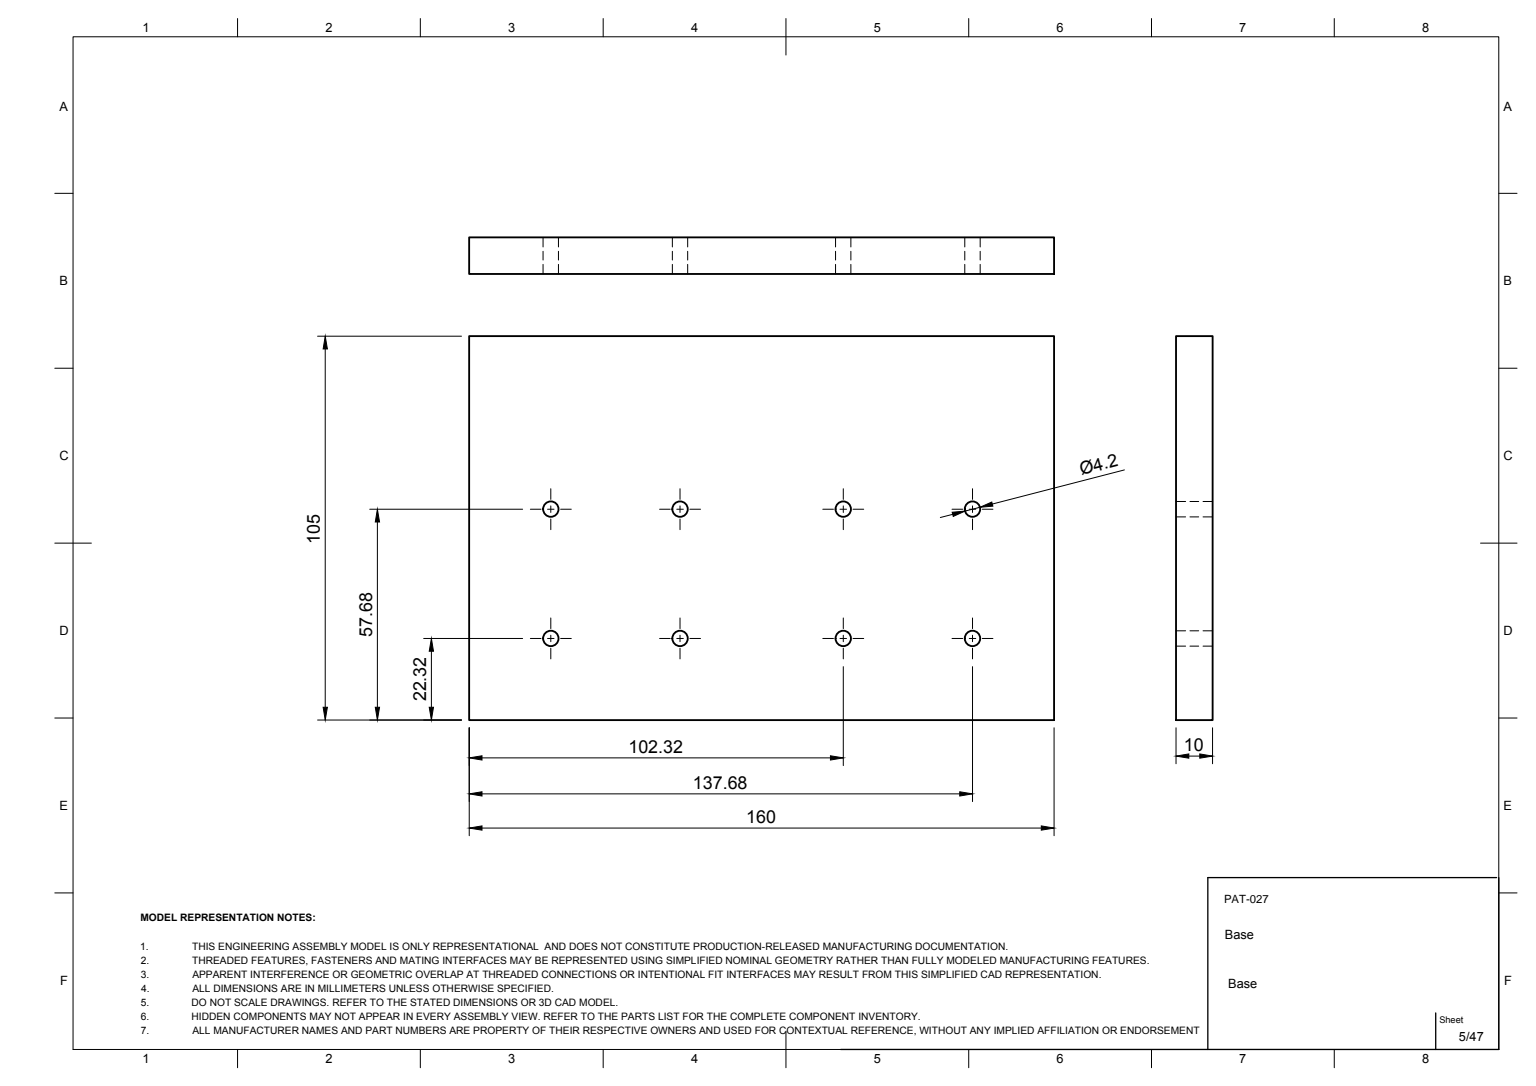
ISO-10303-21;
HEADER;
/* Generated by software containing ST-Developer
 * from STEP Tools, Inc. (www.steptools.com) 
 */

FILE_DESCRIPTION(
/* description */ ('Crank-driven oscillating fan base (mechanism only)'),

/* implementation_level */ '2;1');

FILE_NAME(
/* name */ 'Base.step',
/* time_stamp */ '2026-10-28T03:25:00-07:00',
/* author */ (''),
/* organization */ (''),
/* preprocessor_version */ 'ST-DEVELOPER v20.2',
/* originating_system */ 'Autodesk Translation Framework v15.17.0.0',
/* authorisation */ '');

FILE_SCHEMA (('AUTOMOTIVE_DESIGN { 1 0 10303 214 3 1 1 }'));
ENDSEC;

DATA;
#10=MECHANICAL_DESIGN_GEOMETRIC_PRESENTATION_REPRESENTATION('',(#437),#11916);
#357=SHAPE_REPRESENTATION_RELATIONSHIP('SRR','None',#12081,#397);
#397=ADVANCED_BREP_SHAPE_REPRESENTATION('',(#485),#11872);
#437=STYLED_ITEM('',(#12354),#485);
#485=MANIFOLD_SOLID_BREP('Body1',#6067);
#530=FACE_BOUND('',#1274,.T.);
#531=FACE_BOUND('',#1275,.T.);
#532=FACE_BOUND('',#1276,.T.);
#533=FACE_BOUND('',#1277,.T.);
#534=FACE_BOUND('',#1278,.T.);
#535=FACE_BOUND('',#1279,.T.);
#536=FACE_BOUND('',#1280,.T.);
#537=FACE_BOUND('',#1281,.T.);
#538=FACE_BOUND('',#1283,.T.);
#539=FACE_BOUND('',#1284,.T.);
#540=FACE_BOUND('',#1285,.T.);
#541=FACE_BOUND('',#1286,.T.);
#542=FACE_BOUND('',#1287,.T.);
#543=FACE_BOUND('',#1288,.T.);
#544=FACE_BOUND('',#1289,.T.);
#545=FACE_BOUND('',#1290,.T.);
#692=PLANE('',#6586);
#693=PLANE('',#6587);
#694=PLANE('',#6588);
#695=PLANE('',#6589);
#696=PLANE('',#6590);
#697=PLANE('',#6591);
#886=FACE_OUTER_BOUND('',#1261,.T.);
#887=FACE_OUTER_BOUND('',#1262,.T.);
#888=FACE_OUTER_BOUND('',#1263,.T.);
#889=FACE_OUTER_BOUND('',#1264,.T.);
#890=FACE_OUTER_BOUND('',#1265,.T.);
#891=FACE_OUTER_BOUND('',#1266,.T.);
#892=FACE_OUTER_BOUND('',#1267,.T.);
#893=FACE_OUTER_BOUND('',#1268,.T.);
#894=FACE_OUTER_BOUND('',#1269,.T.);
#895=FACE_OUTER_BOUND('',#1270,.T.);
#896=FACE_OUTER_BOUND('',#1271,.T.);
#897=FACE_OUTER_BOUND('',#1272,.T.);
#898=FACE_OUTER_BOUND('',#1273,.T.);
#899=FACE_OUTER_BOUND('',#1282,.T.);
#1261=EDGE_LOOP('',(#4068,#4069,#4070,#4071));
#1262=EDGE_LOOP('',(#4072,#4073,#4074,#4075));
#1263=EDGE_LOOP('',(#4076,#4077,#4078,#4079));
#1264=EDGE_LOOP('',(#4080,#4081,#4082,#4083));
#1265=EDGE_LOOP('',(#4084,#4085,#4086,#4087));
#1266=EDGE_LOOP('',(#4088,#4089,#4090,#4091));
#1267=EDGE_LOOP('',(#4092,#4093,#4094,#4095));
#1268=EDGE_LOOP('',(#4096,#4097,#4098,#4099));
#1269=EDGE_LOOP('',(#4100,#4101,#4102,#4103));
#1270=EDGE_LOOP('',(#4104,#4105,#4106,#4107));
#1271=EDGE_LOOP('',(#4108,#4109,#4110,#4111));
#1272=EDGE_LOOP('',(#4112,#4113,#4114,#4115));
#1273=EDGE_LOOP('',(#4116,#4117,#4118,#4119));
#1274=EDGE_LOOP('',(#4120));
#1275=EDGE_LOOP('',(#4121));
#1276=EDGE_LOOP('',(#4122));
#1277=EDGE_LOOP('',(#4123));
#1278=EDGE_LOOP('',(#4124));
#1279=EDGE_LOOP('',(#4125));
#1280=EDGE_LOOP('',(#4126));
#1281=EDGE_LOOP('',(#4127));
#1282=EDGE_LOOP('',(#4128,#4129,#4130,#4131));
#1283=EDGE_LOOP('',(#4132));
#1284=EDGE_LOOP('',(#4133));
#1285=EDGE_LOOP('',(#4134));
#1286=EDGE_LOOP('',(#4135));
#1287=EDGE_LOOP('',(#4136));
#1288=EDGE_LOOP('',(#4137));
#1289=EDGE_LOOP('',(#4138));
#1290=EDGE_LOOP('',(#4139));
#1798=LINE('',#9455,#2131);
#1799=LINE('',#9461,#2132);
#1800=LINE('',#9467,#2133);
#1801=LINE('',#9473,#2134);
#1802=LINE('',#9479,#2135);
#1803=LINE('',#9485,#2136);
#1804=LINE('',#9491,#2137);
#1805=LINE('',#9497,#2138);
#1806=LINE('',#9502,#2139);
#1807=LINE('',#9504,#2140);
#1808=LINE('',#9506,#2141);
#1809=LINE('',#9507,#2142);
#1810=LINE('',#9510,#2143);
#1811=LINE('',#9512,#2144);
#1812=LINE('',#9513,#2145);
#1813=LINE('',#9516,#2146);
#1814=LINE('',#9518,#2147);
#1815=LINE('',#9519,#2148);
#1816=LINE('',#9521,#2149);
#1817=LINE('',#9522,#2150);
#2131=VECTOR('',#7421,0.21);
#2132=VECTOR('',#7428,0.21);
#2133=VECTOR('',#7435,0.210000000000001);
#2134=VECTOR('',#7442,0.210000000000001);
#2135=VECTOR('',#7449,0.21);
#2136=VECTOR('',#7456,0.21);
#2137=VECTOR('',#7463,0.21);
#2138=VECTOR('',#7470,0.21);
#2139=VECTOR('',#7475,1.);
#2140=VECTOR('',#7476,1.);
#2141=VECTOR('',#7477,1.);
#2142=VECTOR('',#7478,1.);
#2143=VECTOR('',#7481,1.);
#2144=VECTOR('',#7482,1.);
#2145=VECTOR('',#7483,1.);
#2146=VECTOR('',#7486,1.);
#2147=VECTOR('',#7487,1.);
#2148=VECTOR('',#7488,1.);
#2149=VECTOR('',#7491,1.);
#2150=VECTOR('',#7492,1.);
#2464=CIRCLE('',#6563,0.21);
#2465=CIRCLE('',#6564,0.21);
#2466=CIRCLE('',#6566,0.21);
#2467=CIRCLE('',#6567,0.21);
#2468=CIRCLE('',#6569,0.210000000000001);
#2469=CIRCLE('',#6570,0.210000000000001);
#2470=CIRCLE('',#6572,0.210000000000001);
#2471=CIRCLE('',#6573,0.210000000000001);
#2472=CIRCLE('',#6575,0.21);
#2473=CIRCLE('',#6576,0.21);
#2474=CIRCLE('',#6578,0.21);
#2475=CIRCLE('',#6579,0.21);
#2476=CIRCLE('',#6581,0.21);
#2477=CIRCLE('',#6582,0.21);
#2478=CIRCLE('',#6584,0.21);
#2479=CIRCLE('',#6585,0.21);
#2829=VERTEX_POINT('',#9452);
#2830=VERTEX_POINT('',#9454);
#2831=VERTEX_POINT('',#9458);
#2832=VERTEX_POINT('',#9460);
#2833=VERTEX_POINT('',#9464);
#2834=VERTEX_POINT('',#9466);
#2835=VERTEX_POINT('',#9470);
#2836=VERTEX_POINT('',#9472);
#2837=VERTEX_POINT('',#9476);
#2838=VERTEX_POINT('',#9478);
#2839=VERTEX_POINT('',#9482);
#2840=VERTEX_POINT('',#9484);
#2841=VERTEX_POINT('',#9488);
#2842=VERTEX_POINT('',#9490);
#2843=VERTEX_POINT('',#9494);
#2844=VERTEX_POINT('',#9496);
#2845=VERTEX_POINT('',#9500);
#2846=VERTEX_POINT('',#9501);
#2847=VERTEX_POINT('',#9503);
#2848=VERTEX_POINT('',#9505);
#2849=VERTEX_POINT('',#9509);
#2850=VERTEX_POINT('',#9511);
#2851=VERTEX_POINT('',#9515);
#2852=VERTEX_POINT('',#9517);
#3329=EDGE_CURVE('',#2829,#2829,#2464,.T.);
#3330=EDGE_CURVE('',#2829,#2830,#1798,.T.);
#3331=EDGE_CURVE('',#2830,#2830,#2465,.T.);
#3332=EDGE_CURVE('',#2831,#2831,#2466,.T.);
#3333=EDGE_CURVE('',#2831,#2832,#1799,.T.);
#3334=EDGE_CURVE('',#2832,#2832,#2467,.T.);
#3335=EDGE_CURVE('',#2833,#2833,#2468,.T.);
#3336=EDGE_CURVE('',#2833,#2834,#1800,.T.);
#3337=EDGE_CURVE('',#2834,#2834,#2469,.T.);
#3338=EDGE_CURVE('',#2835,#2835,#2470,.T.);
#3339=EDGE_CURVE('',#2835,#2836,#1801,.T.);
#3340=EDGE_CURVE('',#2836,#2836,#2471,.T.);
#3341=EDGE_CURVE('',#2837,#2837,#2472,.T.);
#3342=EDGE_CURVE('',#2837,#2838,#1802,.T.);
#3343=EDGE_CURVE('',#2838,#2838,#2473,.T.);
#3344=EDGE_CURVE('',#2839,#2839,#2474,.T.);
#3345=EDGE_CURVE('',#2839,#2840,#1803,.T.);
#3346=EDGE_CURVE('',#2840,#2840,#2475,.T.);
#3347=EDGE_CURVE('',#2841,#2841,#2476,.T.);
#3348=EDGE_CURVE('',#2841,#2842,#1804,.T.);
#3349=EDGE_CURVE('',#2842,#2842,#2477,.T.);
#3350=EDGE_CURVE('',#2843,#2843,#2478,.T.);
#3351=EDGE_CURVE('',#2843,#2844,#1805,.T.);
#3352=EDGE_CURVE('',#2844,#2844,#2479,.T.);
#3353=EDGE_CURVE('',#2845,#2846,#1806,.T.);
#3354=EDGE_CURVE('',#2846,#2847,#1807,.T.);
#3355=EDGE_CURVE('',#2848,#2847,#1808,.T.);
#3356=EDGE_CURVE('',#2845,#2848,#1809,.T.);
#3357=EDGE_CURVE('',#2849,#2845,#1810,.T.);
#3358=EDGE_CURVE('',#2850,#2848,#1811,.T.);
#3359=EDGE_CURVE('',#2849,#2850,#1812,.T.);
#3360=EDGE_CURVE('',#2851,#2849,#1813,.T.);
#3361=EDGE_CURVE('',#2852,#2850,#1814,.T.);
#3362=EDGE_CURVE('',#2851,#2852,#1815,.T.);
#3363=EDGE_CURVE('',#2846,#2851,#1816,.T.);
#3364=EDGE_CURVE('',#2847,#2852,#1817,.T.);
#4068=ORIENTED_EDGE('',*,*,#3329,.F.);
#4069=ORIENTED_EDGE('',*,*,#3330,.T.);
#4070=ORIENTED_EDGE('',*,*,#3331,.F.);
#4071=ORIENTED_EDGE('',*,*,#3330,.F.);
#4072=ORIENTED_EDGE('',*,*,#3332,.F.);
#4073=ORIENTED_EDGE('',*,*,#3333,.T.);
#4074=ORIENTED_EDGE('',*,*,#3334,.F.);
#4075=ORIENTED_EDGE('',*,*,#3333,.F.);
#4076=ORIENTED_EDGE('',*,*,#3335,.F.);
#4077=ORIENTED_EDGE('',*,*,#3336,.T.);
#4078=ORIENTED_EDGE('',*,*,#3337,.F.);
#4079=ORIENTED_EDGE('',*,*,#3336,.F.);
#4080=ORIENTED_EDGE('',*,*,#3338,.F.);
#4081=ORIENTED_EDGE('',*,*,#3339,.T.);
#4082=ORIENTED_EDGE('',*,*,#3340,.F.);
#4083=ORIENTED_EDGE('',*,*,#3339,.F.);
#4084=ORIENTED_EDGE('',*,*,#3341,.F.);
#4085=ORIENTED_EDGE('',*,*,#3342,.T.);
#4086=ORIENTED_EDGE('',*,*,#3343,.F.);
#4087=ORIENTED_EDGE('',*,*,#3342,.F.);
#4088=ORIENTED_EDGE('',*,*,#3344,.F.);
#4089=ORIENTED_EDGE('',*,*,#3345,.T.);
#4090=ORIENTED_EDGE('',*,*,#3346,.F.);
#4091=ORIENTED_EDGE('',*,*,#3345,.F.);
#4092=ORIENTED_EDGE('',*,*,#3347,.F.);
#4093=ORIENTED_EDGE('',*,*,#3348,.T.);
#4094=ORIENTED_EDGE('',*,*,#3349,.F.);
#4095=ORIENTED_EDGE('',*,*,#3348,.F.);
#4096=ORIENTED_EDGE('',*,*,#3350,.F.);
#4097=ORIENTED_EDGE('',*,*,#3351,.T.);
#4098=ORIENTED_EDGE('',*,*,#3352,.F.);
#4099=ORIENTED_EDGE('',*,*,#3351,.F.);
#4100=ORIENTED_EDGE('',*,*,#3353,.T.);
#4101=ORIENTED_EDGE('',*,*,#3354,.T.);
#4102=ORIENTED_EDGE('',*,*,#3355,.F.);
#4103=ORIENTED_EDGE('',*,*,#3356,.F.);
#4104=ORIENTED_EDGE('',*,*,#3357,.T.);
#4105=ORIENTED_EDGE('',*,*,#3356,.T.);
#4106=ORIENTED_EDGE('',*,*,#3358,.F.);
#4107=ORIENTED_EDGE('',*,*,#3359,.F.);
#4108=ORIENTED_EDGE('',*,*,#3360,.T.);
#4109=ORIENTED_EDGE('',*,*,#3359,.T.);
#4110=ORIENTED_EDGE('',*,*,#3361,.F.);
#4111=ORIENTED_EDGE('',*,*,#3362,.F.);
#4112=ORIENTED_EDGE('',*,*,#3363,.T.);
#4113=ORIENTED_EDGE('',*,*,#3362,.T.);
#4114=ORIENTED_EDGE('',*,*,#3364,.F.);
#4115=ORIENTED_EDGE('',*,*,#3354,.F.);
#4116=ORIENTED_EDGE('',*,*,#3364,.T.);
#4117=ORIENTED_EDGE('',*,*,#3361,.T.);
#4118=ORIENTED_EDGE('',*,*,#3358,.T.);
#4119=ORIENTED_EDGE('',*,*,#3355,.T.);
#4120=ORIENTED_EDGE('',*,*,#3352,.T.);
#4121=ORIENTED_EDGE('',*,*,#3349,.T.);
#4122=ORIENTED_EDGE('',*,*,#3346,.T.);
#4123=ORIENTED_EDGE('',*,*,#3343,.T.);
#4124=ORIENTED_EDGE('',*,*,#3340,.T.);
#4125=ORIENTED_EDGE('',*,*,#3337,.T.);
#4126=ORIENTED_EDGE('',*,*,#3334,.T.);
#4127=ORIENTED_EDGE('',*,*,#3331,.T.);
#4128=ORIENTED_EDGE('',*,*,#3363,.F.);
#4129=ORIENTED_EDGE('',*,*,#3353,.F.);
#4130=ORIENTED_EDGE('',*,*,#3357,.F.);
#4131=ORIENTED_EDGE('',*,*,#3360,.F.);
#4132=ORIENTED_EDGE('',*,*,#3350,.T.);
#4133=ORIENTED_EDGE('',*,*,#3347,.T.);
#4134=ORIENTED_EDGE('',*,*,#3344,.T.);
#4135=ORIENTED_EDGE('',*,*,#3341,.T.);
#4136=ORIENTED_EDGE('',*,*,#3338,.T.);
#4137=ORIENTED_EDGE('',*,*,#3335,.T.);
#4138=ORIENTED_EDGE('',*,*,#3332,.T.);
#4139=ORIENTED_EDGE('',*,*,#3329,.T.);
#5546=CYLINDRICAL_SURFACE('',#6562,0.21);
#5547=CYLINDRICAL_SURFACE('',#6565,0.21);
#5548=CYLINDRICAL_SURFACE('',#6568,0.210000000000001);
#5549=CYLINDRICAL_SURFACE('',#6571,0.210000000000001);
#5550=CYLINDRICAL_SURFACE('',#6574,0.21);
#5551=CYLINDRICAL_SURFACE('',#6577,0.21);
#5552=CYLINDRICAL_SURFACE('',#6580,0.21);
#5553=CYLINDRICAL_SURFACE('',#6583,0.21);
#5692=ADVANCED_FACE('',(#886),#5546,.F.);
#5693=ADVANCED_FACE('',(#887),#5547,.F.);
#5694=ADVANCED_FACE('',(#888),#5548,.F.);
#5695=ADVANCED_FACE('',(#889),#5549,.F.);
#5696=ADVANCED_FACE('',(#890),#5550,.F.);
#5697=ADVANCED_FACE('',(#891),#5551,.F.);
#5698=ADVANCED_FACE('',(#892),#5552,.F.);
#5699=ADVANCED_FACE('',(#893),#5553,.F.);
#5700=ADVANCED_FACE('',(#894),#692,.T.);
#5701=ADVANCED_FACE('',(#895),#693,.T.);
#5702=ADVANCED_FACE('',(#896),#694,.T.);
#5703=ADVANCED_FACE('',(#897),#695,.T.);
#5704=ADVANCED_FACE('',(#898,#530,#531,#532,#533,#534,#535,#536,#537),#696,
 .T.);
#5705=ADVANCED_FACE('',(#899,#538,#539,#540,#541,#542,#543,#544,#545),#697,
 .F.);
#6067=CLOSED_SHELL('',(#5692,#5693,#5694,#5695,#5696,#5697,#5698,#5699,
#5700,#5701,#5702,#5703,#5704,#5705));
#6561=AXIS2_PLACEMENT_3D('',#9450,#7415,#7416);
#6562=AXIS2_PLACEMENT_3D('',#9451,#7417,#7418);
#6563=AXIS2_PLACEMENT_3D('',#9453,#7419,#7420);
#6564=AXIS2_PLACEMENT_3D('',#9456,#7422,#7423);
#6565=AXIS2_PLACEMENT_3D('',#9457,#7424,#7425);
#6566=AXIS2_PLACEMENT_3D('',#9459,#7426,#7427);
#6567=AXIS2_PLACEMENT_3D('',#9462,#7429,#7430);
#6568=AXIS2_PLACEMENT_3D('',#9463,#7431,#7432);
#6569=AXIS2_PLACEMENT_3D('',#9465,#7433,#7434);
#6570=AXIS2_PLACEMENT_3D('',#9468,#7436,#7437);
#6571=AXIS2_PLACEMENT_3D('',#9469,#7438,#7439);
#6572=AXIS2_PLACEMENT_3D('',#9471,#7440,#7441);
#6573=AXIS2_PLACEMENT_3D('',#9474,#7443,#7444);
#6574=AXIS2_PLACEMENT_3D('',#9475,#7445,#7446);
#6575=AXIS2_PLACEMENT_3D('',#9477,#7447,#7448);
#6576=AXIS2_PLACEMENT_3D('',#9480,#7450,#7451);
#6577=AXIS2_PLACEMENT_3D('',#9481,#7452,#7453);
#6578=AXIS2_PLACEMENT_3D('',#9483,#7454,#7455);
#6579=AXIS2_PLACEMENT_3D('',#9486,#7457,#7458);
#6580=AXIS2_PLACEMENT_3D('',#9487,#7459,#7460);
#6581=AXIS2_PLACEMENT_3D('',#9489,#7461,#7462);
#6582=AXIS2_PLACEMENT_3D('',#9492,#7464,#7465);
#6583=AXIS2_PLACEMENT_3D('',#9493,#7466,#7467);
#6584=AXIS2_PLACEMENT_3D('',#9495,#7468,#7469);
#6585=AXIS2_PLACEMENT_3D('',#9498,#7471,#7472);
#6586=AXIS2_PLACEMENT_3D('',#9499,#7473,#7474);
#6587=AXIS2_PLACEMENT_3D('',#9508,#7479,#7480);
#6588=AXIS2_PLACEMENT_3D('',#9514,#7484,#7485);
#6589=AXIS2_PLACEMENT_3D('',#9520,#7489,#7490);
#6590=AXIS2_PLACEMENT_3D('',#9523,#7493,#7494);
#6591=AXIS2_PLACEMENT_3D('',#9524,#7495,#7496);
#7415=DIRECTION('axis',(0.,0.,1.));
#7416=DIRECTION('refdir',(1.,0.,0.));
#7417=DIRECTION('center_axis',(0.,0.,1.));
#7418=DIRECTION('ref_axis',(1.,0.,0.));
#7419=DIRECTION('center_axis',(0.,0.,1.));
#7420=DIRECTION('ref_axis',(1.,0.,0.));
#7421=DIRECTION('',(0.,0.,1.));
#7422=DIRECTION('center_axis',(0.,0.,-1.));
#7423=DIRECTION('ref_axis',(1.,0.,0.));
#7424=DIRECTION('center_axis',(0.,0.,1.));
#7425=DIRECTION('ref_axis',(1.,0.,0.));
#7426=DIRECTION('center_axis',(0.,0.,1.));
#7427=DIRECTION('ref_axis',(1.,0.,0.));
#7428=DIRECTION('',(0.,0.,1.));
#7429=DIRECTION('center_axis',(0.,0.,-1.));
#7430=DIRECTION('ref_axis',(1.,0.,0.));
#7431=DIRECTION('center_axis',(0.,0.,1.));
#7432=DIRECTION('ref_axis',(1.,0.,0.));
#7433=DIRECTION('center_axis',(0.,0.,1.));
#7434=DIRECTION('ref_axis',(1.,0.,0.));
#7435=DIRECTION('',(0.,0.,1.));
#7436=DIRECTION('center_axis',(0.,0.,-1.));
#7437=DIRECTION('ref_axis',(1.,0.,0.));
#7438=DIRECTION('center_axis',(0.,0.,1.));
#7439=DIRECTION('ref_axis',(1.,0.,0.));
#7440=DIRECTION('center_axis',(0.,0.,1.));
#7441=DIRECTION('ref_axis',(1.,0.,0.));
#7442=DIRECTION('',(0.,0.,1.));
#7443=DIRECTION('center_axis',(0.,0.,-1.));
#7444=DIRECTION('ref_axis',(1.,0.,0.));
#7445=DIRECTION('center_axis',(0.,0.,1.));
#7446=DIRECTION('ref_axis',(1.,0.,0.));
#7447=DIRECTION('center_axis',(0.,0.,1.));
#7448=DIRECTION('ref_axis',(1.,0.,0.));
#7449=DIRECTION('',(0.,0.,1.));
#7450=DIRECTION('center_axis',(0.,0.,-1.));
#7451=DIRECTION('ref_axis',(1.,0.,0.));
#7452=DIRECTION('center_axis',(0.,0.,1.));
#7453=DIRECTION('ref_axis',(1.,0.,0.));
#7454=DIRECTION('center_axis',(0.,0.,1.));
#7455=DIRECTION('ref_axis',(1.,0.,0.));
#7456=DIRECTION('',(0.,0.,1.));
#7457=DIRECTION('center_axis',(0.,0.,-1.));
#7458=DIRECTION('ref_axis',(1.,0.,0.));
#7459=DIRECTION('center_axis',(0.,0.,1.));
#7460=DIRECTION('ref_axis',(1.,0.,0.));
#7461=DIRECTION('center_axis',(0.,0.,1.));
#7462=DIRECTION('ref_axis',(1.,0.,0.));
#7463=DIRECTION('',(0.,0.,1.));
#7464=DIRECTION('center_axis',(0.,0.,-1.));
#7465=DIRECTION('ref_axis',(1.,0.,0.));
#7466=DIRECTION('center_axis',(0.,0.,1.));
#7467=DIRECTION('ref_axis',(1.,0.,0.));
#7468=DIRECTION('center_axis',(0.,0.,1.));
#7469=DIRECTION('ref_axis',(1.,0.,0.));
#7470=DIRECTION('',(0.,0.,1.));
#7471=DIRECTION('center_axis',(0.,0.,-1.));
#7472=DIRECTION('ref_axis',(1.,0.,0.));
#7473=DIRECTION('center_axis',(0.,1.,0.));
#7474=DIRECTION('ref_axis',(-1.,0.,0.));
#7475=DIRECTION('',(-1.,0.,0.));
#7476=DIRECTION('',(0.,0.,1.));
#7477=DIRECTION('',(-1.,0.,0.));
#7478=DIRECTION('',(0.,0.,1.));
#7479=DIRECTION('center_axis',(1.,0.,0.));
#7480=DIRECTION('ref_axis',(0.,1.,0.));
#7481=DIRECTION('',(0.,1.,0.));
#7482=DIRECTION('',(0.,1.,0.));
#7483=DIRECTION('',(0.,0.,1.));
#7484=DIRECTION('center_axis',(0.,-1.,0.));
#7485=DIRECTION('ref_axis',(1.,0.,0.));
#7486=DIRECTION('',(1.,0.,0.));
#7487=DIRECTION('',(1.,0.,0.));
#7488=DIRECTION('',(0.,0.,1.));
#7489=DIRECTION('center_axis',(-1.,0.,0.));
#7490=DIRECTION('ref_axis',(0.,-1.,0.));
#7491=DIRECTION('',(0.,-1.,0.));
#7492=DIRECTION('',(0.,-1.,0.));
#7493=DIRECTION('center_axis',(0.,0.,1.));
#7494=DIRECTION('ref_axis',(1.,0.,0.));
#7495=DIRECTION('center_axis',(0.,0.,1.));
#7496=DIRECTION('ref_axis',(1.,0.,0.));
#9450=CARTESIAN_POINT('',(0.,0.,0.));
#9451=CARTESIAN_POINT('Origin',(6.23223304703363,-1.76776695296637,-0.1));
#9452=CARTESIAN_POINT('',(6.02223304703363,-1.76776695296637,0.));
#9453=CARTESIAN_POINT('Origin',(6.23223304703363,-1.76776695296637,0.));
#9454=CARTESIAN_POINT('',(6.02223304703363,-1.76776695296637,1.));
#9455=CARTESIAN_POINT('',(6.02223304703363,-1.76776695296637,-0.1));
#9456=CARTESIAN_POINT('Origin',(6.23223304703363,-1.76776695296637,1.));
#9457=CARTESIAN_POINT('Origin',(6.23223304703363,1.76776695296637,-0.1));
#9458=CARTESIAN_POINT('',(6.02223304703363,1.76776695296637,0.));
#9459=CARTESIAN_POINT('Origin',(6.23223304703363,1.76776695296637,0.));
#9460=CARTESIAN_POINT('',(6.02223304703363,1.76776695296637,1.));
#9461=CARTESIAN_POINT('',(6.02223304703363,1.76776695296637,-0.1));
#9462=CARTESIAN_POINT('Origin',(6.23223304703363,1.76776695296637,1.));
#9463=CARTESIAN_POINT('Origin',(9.76776695296637,1.76776695296637,-0.1));
#9464=CARTESIAN_POINT('',(9.55776695296637,1.76776695296637,0.));
#9465=CARTESIAN_POINT('Origin',(9.76776695296637,1.76776695296637,0.));
#9466=CARTESIAN_POINT('',(9.55776695296637,1.76776695296637,1.));
#9467=CARTESIAN_POINT('',(9.55776695296637,1.76776695296637,-0.1));
#9468=CARTESIAN_POINT('Origin',(9.76776695296637,1.76776695296637,1.));
#9469=CARTESIAN_POINT('Origin',(9.76776695296637,-1.76776695296637,-0.1));
#9470=CARTESIAN_POINT('',(9.55776695296637,-1.76776695296637,0.));
#9471=CARTESIAN_POINT('Origin',(9.76776695296637,-1.76776695296637,0.));
#9472=CARTESIAN_POINT('',(9.55776695296637,-1.76776695296637,1.));
#9473=CARTESIAN_POINT('',(9.55776695296637,-1.76776695296637,-0.1));
#9474=CARTESIAN_POINT('Origin',(9.76776695296637,-1.76776695296637,1.));
#9475=CARTESIAN_POINT('Origin',(-1.76776695296637,-1.76776695296637,-0.1));
#9476=CARTESIAN_POINT('',(-1.97776695296637,-1.76776695296637,0.));
#9477=CARTESIAN_POINT('Origin',(-1.76776695296637,-1.76776695296637,0.));
#9478=CARTESIAN_POINT('',(-1.97776695296637,-1.76776695296637,1.));
#9479=CARTESIAN_POINT('',(-1.97776695296637,-1.76776695296637,-0.1));
#9480=CARTESIAN_POINT('Origin',(-1.76776695296637,-1.76776695296637,1.));
#9481=CARTESIAN_POINT('Origin',(-1.76776695296637,1.76776695296637,-0.1));
#9482=CARTESIAN_POINT('',(-1.97776695296637,1.76776695296637,0.));
#9483=CARTESIAN_POINT('Origin',(-1.76776695296637,1.76776695296637,0.));
#9484=CARTESIAN_POINT('',(-1.97776695296637,1.76776695296637,1.));
#9485=CARTESIAN_POINT('',(-1.97776695296637,1.76776695296637,-0.1));
#9486=CARTESIAN_POINT('Origin',(-1.76776695296637,1.76776695296637,1.));
#9487=CARTESIAN_POINT('Origin',(1.76776695296637,1.76776695296637,-0.1));
#9488=CARTESIAN_POINT('',(1.55776695296637,1.76776695296637,0.));
#9489=CARTESIAN_POINT('Origin',(1.76776695296637,1.76776695296637,0.));
#9490=CARTESIAN_POINT('',(1.55776695296637,1.76776695296637,1.));
#9491=CARTESIAN_POINT('',(1.55776695296637,1.76776695296637,-0.1));
#9492=CARTESIAN_POINT('Origin',(1.76776695296637,1.76776695296637,1.));
#9493=CARTESIAN_POINT('Origin',(1.76776695296637,-1.76776695296637,-0.1));
#9494=CARTESIAN_POINT('',(1.55776695296637,-1.76776695296637,0.));
#9495=CARTESIAN_POINT('Origin',(1.76776695296637,-1.76776695296637,0.));
#9496=CARTESIAN_POINT('',(1.55776695296637,-1.76776695296637,1.));
#9497=CARTESIAN_POINT('',(1.55776695296637,-1.76776695296637,-0.1));
#9498=CARTESIAN_POINT('Origin',(1.76776695296637,-1.76776695296637,1.));
#9499=CARTESIAN_POINT('Origin',(12.,6.5,0.));
#9500=CARTESIAN_POINT('',(12.,6.5,0.));
#9501=CARTESIAN_POINT('',(-4.,6.5,0.));
#9502=CARTESIAN_POINT('',(12.,6.5,0.));
#9503=CARTESIAN_POINT('',(-4.,6.5,1.));
#9504=CARTESIAN_POINT('',(-4.,6.5,0.));
#9505=CARTESIAN_POINT('',(12.,6.5,1.));
#9506=CARTESIAN_POINT('',(12.,6.5,1.));
#9507=CARTESIAN_POINT('',(12.,6.5,0.));
#9508=CARTESIAN_POINT('Origin',(12.,-4.,0.));
#9509=CARTESIAN_POINT('',(12.,-4.,0.));
#9510=CARTESIAN_POINT('',(12.,-4.,0.));
#9511=CARTESIAN_POINT('',(12.,-4.,1.));
#9512=CARTESIAN_POINT('',(12.,-4.,1.));
#9513=CARTESIAN_POINT('',(12.,-4.,0.));
#9514=CARTESIAN_POINT('Origin',(-4.,-4.,0.));
#9515=CARTESIAN_POINT('',(-4.,-4.,0.));
#9516=CARTESIAN_POINT('',(-4.,-4.,0.));
#9517=CARTESIAN_POINT('',(-4.,-4.,1.));
#9518=CARTESIAN_POINT('',(-4.,-4.,1.));
#9519=CARTESIAN_POINT('',(-4.,-4.,0.));
#9520=CARTESIAN_POINT('Origin',(-4.,6.5,0.));
#9521=CARTESIAN_POINT('',(-4.,6.5,0.));
#9522=CARTESIAN_POINT('',(-4.,6.5,1.));
#9523=CARTESIAN_POINT('Origin',(4.,1.25,1.));
#9524=CARTESIAN_POINT('Origin',(4.,1.25,0.));
#11825=UNCERTAINTY_MEASURE_WITH_UNIT(LENGTH_MEASURE(0.001),#11917,
'DISTANCE_ACCURACY_VALUE',
'Maximum model space distance between geometric entities at asserted c
onnectivities');
#11869=UNCERTAINTY_MEASURE_WITH_UNIT(LENGTH_MEASURE(0.001),#11917,
'DISTANCE_ACCURACY_VALUE',
'Maximum model space distance between geometric entities at asserted c
onnectivities');
#11872=(
GEOMETRIC_REPRESENTATION_CONTEXT(3)
GLOBAL_UNCERTAINTY_ASSIGNED_CONTEXT((#11825))
GLOBAL_UNIT_ASSIGNED_CONTEXT((#11917,#11919,#11920))
REPRESENTATION_CONTEXT('','3D')
);
#11916=(
GEOMETRIC_REPRESENTATION_CONTEXT(3)
GLOBAL_UNCERTAINTY_ASSIGNED_CONTEXT((#11869))
GLOBAL_UNIT_ASSIGNED_CONTEXT((#11917,#11919,#11920))
REPRESENTATION_CONTEXT('','3D')
);
#11917=(
LENGTH_UNIT()
NAMED_UNIT(*)
SI_UNIT(.CENTI.,.METRE.)
);
#11919=(
NAMED_UNIT(*)
PLANE_ANGLE_UNIT()
SI_UNIT($,.RADIAN.)
);
#11920=(
NAMED_UNIT(*)
SI_UNIT($,.STERADIAN.)
SOLID_ANGLE_UNIT()
);
#11923=SHAPE_DEFINITION_REPRESENTATION(#11969,#12081);
#11969=PRODUCT_DEFINITION_SHAPE('',$,#12128);
#12081=SHAPE_REPRESENTATION('',(#6561),#11872);
#12125=PRODUCT_DEFINITION_CONTEXT('part definition',#12265,'design');
#12128=PRODUCT_DEFINITION('Base','Base',#12174,#12125);
#12174=PRODUCT_DEFINITION_FORMATION('',$,#12269);
#12265=APPLICATION_CONTEXT(
'Core Data for Automotive Mechanical Design Process');
#12266=PRODUCT_CONTEXT('part definition',#12265,'mechanical');
#12269=PRODUCT('Base','Base','Base',(#12266));
#12348=COLOUR_RGB('Dark Blue',0.08,0.2,0.34);
#12349=FILL_AREA_STYLE_COLOUR('',#12348);
#12350=FILL_AREA_STYLE('',(#12349));
#12351=SURFACE_STYLE_FILL_AREA(#12350);
#12352=SURFACE_SIDE_STYLE('',(#12351));
#12353=SURFACE_STYLE_USAGE(.BOTH.,#12352);
#12354=PRESENTATION_STYLE_ASSIGNMENT((#12353));
ENDSEC;
END-ISO-10303-21;
